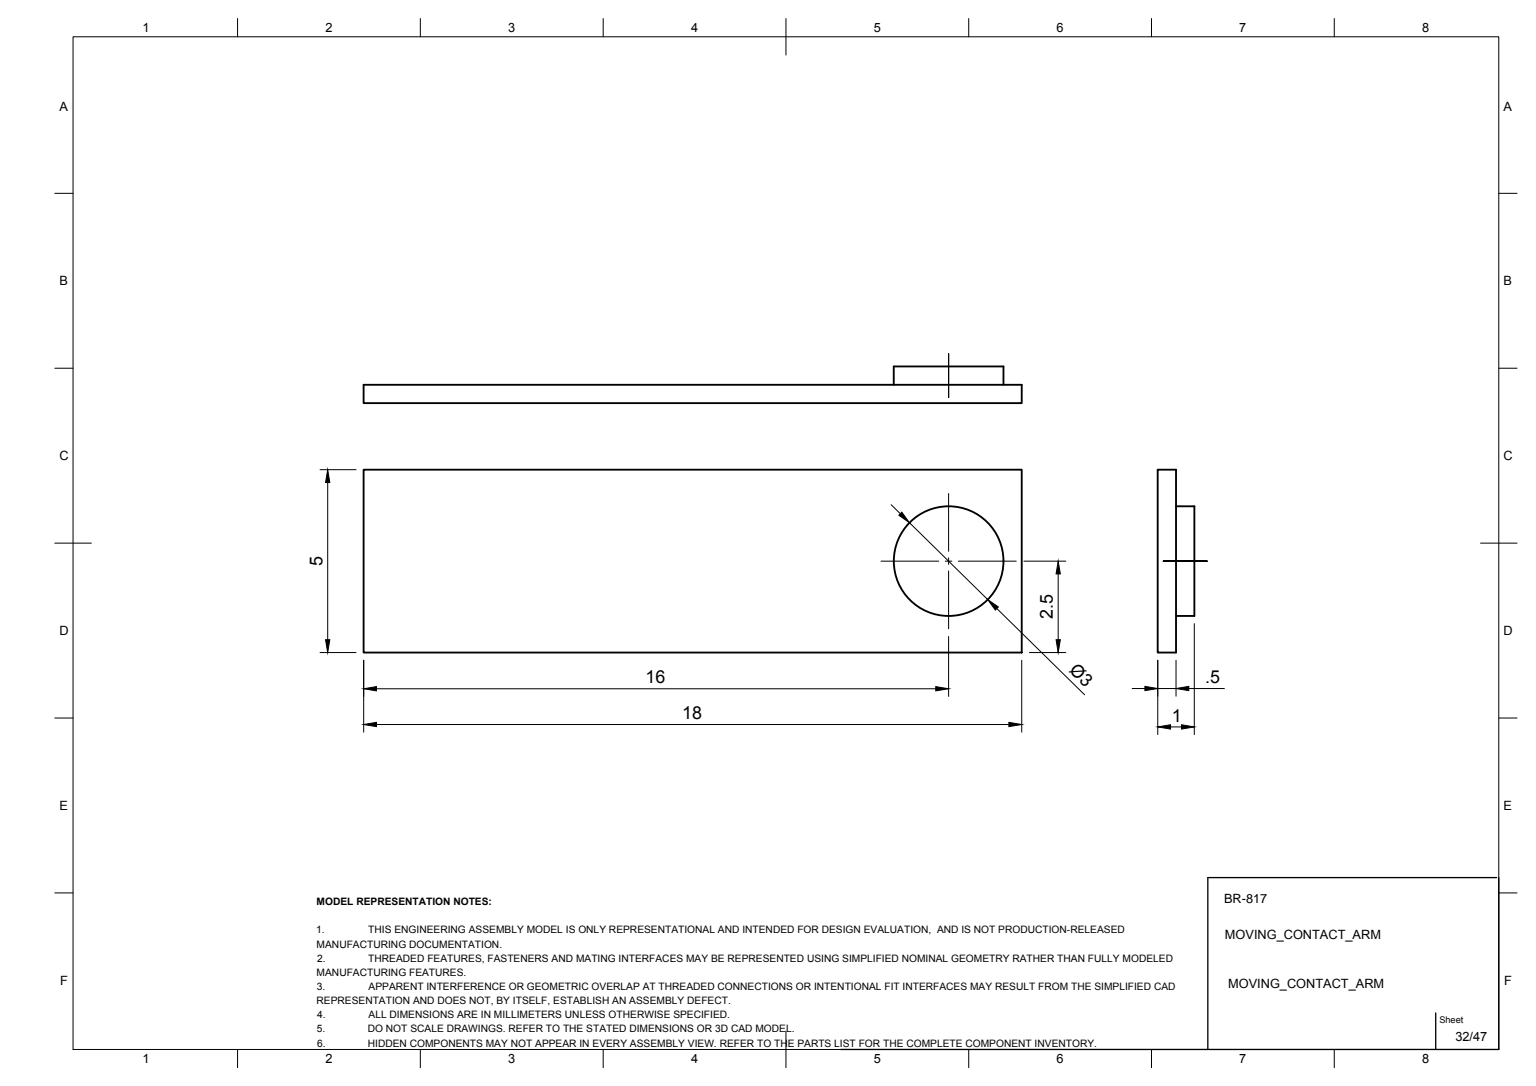
ISO-10303-21;
HEADER;
FILE_DESCRIPTION((''),'2;1');
FILE_NAME('MOVING_CONTACT_ARM.step','2026-10-01T22:07:29-07:00',(''),(''),'','','');
FILE_SCHEMA (('AUTOMOTIVE_DESIGN { 1 0 10303 214 3 1 1 }'));
ENDSEC;
DATA;
#10=MECHANICAL_DESIGN_GEOMETRIC_PRESENTATION_REPRESENTATION('',(#564),#15484);
#494=SHAPE_REPRESENTATION_RELATIONSHIP('SRR','None',#15644,#529) ;
#529=ADVANCED_BREP_SHAPE_REPRESENTATION('',(#605),#15468) ;
#564=STYLED_ITEM('',(#15834),#605) ;
#605=MANIFOLD_SOLID_BREP('MOVING_CONTACT_ARM',#8275) ;
#756=CYLINDRICAL_SURFACE('',#9515,0.15) ;
#875=FACE_BOUND('',#2272,.T.) ;
#1219=CIRCLE('',#9516,0.15) ;
#1220=CIRCLE('',#9517,0.15) ;
#1704=FACE_OUTER_BOUND('',#2269,.T.) ;
#1705=FACE_OUTER_BOUND('',#2270,.T.) ;
#1706=FACE_OUTER_BOUND('',#2271,.T.) ;
#1707=FACE_OUTER_BOUND('',#2273,.T.) ;
#1708=FACE_OUTER_BOUND('',#2274,.T.) ;
#1709=FACE_OUTER_BOUND('',#2275,.T.) ;
#1710=FACE_OUTER_BOUND('',#2276,.T.) ;
#1711=FACE_OUTER_BOUND('',#2277,.T.) ;
#2269=EDGE_LOOP('',(#6843,#6844,#6845,#6846)) ;
#2270=EDGE_LOOP('',(#6847)) ;
#2271=EDGE_LOOP('',(#6848,#6849,#6850,#6851)) ;
#2272=EDGE_LOOP('',(#6852)) ;
#2273=EDGE_LOOP('',(#6853,#6854,#6855,#6856)) ;
#2274=EDGE_LOOP('',(#6857,#6858,#6859,#6860)) ;
#2275=EDGE_LOOP('',(#6861,#6862,#6863,#6864)) ;
#2276=EDGE_LOOP('',(#6865,#6866,#6867,#6868)) ;
#2277=EDGE_LOOP('',(#6869,#6870,#6871,#6872)) ;
#2771=LINE('',#14620,#3245) ;
#2772=LINE('',#14626,#3246) ;
#2773=LINE('',#14628,#3247) ;
#2774=LINE('',#14630,#3248) ;
#2775=LINE('',#14631,#3249) ;
#2776=LINE('',#14635,#3250) ;
#2777=LINE('',#14637,#3251) ;
#2778=LINE('',#14639,#3252) ;
#2779=LINE('',#14640,#3253) ;
#2780=LINE('',#14642,#3254) ;
#2781=LINE('',#14643,#3255) ;
#2782=LINE('',#14645,#3256) ;
#2783=LINE('',#14647,#3257) ;
#3245=VECTOR('',#11926,0.15) ;
#3246=VECTOR('',#11933,1.) ;
#3247=VECTOR('',#11934,1.) ;
#3248=VECTOR('',#11935,1.) ;
#3249=VECTOR('',#11936,1.) ;
#3250=VECTOR('',#11939,1.) ;
#3251=VECTOR('',#11940,1.) ;
#3252=VECTOR('',#11941,1.) ;
#3253=VECTOR('',#11942,1.) ;
#3254=VECTOR('',#11945,1.) ;
#3255=VECTOR('',#11946,1.) ;
#3256=VECTOR('',#11949,1.) ;
#3257=VECTOR('',#11952,1.) ;
#3911=VERTEX_POINT('',#14617) ;
#3912=VERTEX_POINT('',#14619) ;
#3913=VERTEX_POINT('',#14624) ;
#3914=VERTEX_POINT('',#14625) ;
#3915=VERTEX_POINT('',#14627) ;
#3916=VERTEX_POINT('',#14629) ;
#3917=VERTEX_POINT('',#14633) ;
#3918=VERTEX_POINT('',#14634) ;
#3919=VERTEX_POINT('',#14636) ;
#3920=VERTEX_POINT('',#14638) ;
#4926=EDGE_CURVE('',#3911,#3911,#1219,.T.) ;
#4927=EDGE_CURVE('',#3911,#3912,#2771,.T.) ;
#4928=EDGE_CURVE('',#3912,#3912,#1220,.T.) ;
#4929=EDGE_CURVE('',#3913,#3914,#2772,.T.) ;
#4930=EDGE_CURVE('',#3914,#3915,#2773,.T.) ;
#4931=EDGE_CURVE('',#3915,#3916,#2774,.T.) ;
#4932=EDGE_CURVE('',#3916,#3913,#2775,.T.) ;
#4933=EDGE_CURVE('',#3917,#3918,#2776,.T.) ;
#4934=EDGE_CURVE('',#3918,#3919,#2777,.T.) ;
#4935=EDGE_CURVE('',#3919,#3920,#2778,.T.) ;
#4936=EDGE_CURVE('',#3920,#3917,#2779,.T.) ;
#4937=EDGE_CURVE('',#3916,#3919,#2780,.T.) ;
#4938=EDGE_CURVE('',#3913,#3918,#2781,.T.) ;
#4939=EDGE_CURVE('',#3915,#3920,#2782,.T.) ;
#4940=EDGE_CURVE('',#3914,#3917,#2783,.T.) ;
#6843=ORIENTED_EDGE('',*,*,#4926,.F.) ;
#6844=ORIENTED_EDGE('',*,*,#4927,.T.) ;
#6845=ORIENTED_EDGE('',*,*,#4928,.F.) ;
#6846=ORIENTED_EDGE('',*,*,#4927,.F.) ;
#6847=ORIENTED_EDGE('',*,*,#4926,.T.) ;
#6848=ORIENTED_EDGE('',*,*,#4929,.T.) ;
#6849=ORIENTED_EDGE('',*,*,#4930,.T.) ;
#6850=ORIENTED_EDGE('',*,*,#4931,.T.) ;
#6851=ORIENTED_EDGE('',*,*,#4932,.T.) ;
#6852=ORIENTED_EDGE('',*,*,#4928,.T.) ;
#6853=ORIENTED_EDGE('',*,*,#4933,.T.) ;
#6854=ORIENTED_EDGE('',*,*,#4934,.T.) ;
#6855=ORIENTED_EDGE('',*,*,#4935,.T.) ;
#6856=ORIENTED_EDGE('',*,*,#4936,.T.) ;
#6857=ORIENTED_EDGE('',*,*,#4937,.T.) ;
#6858=ORIENTED_EDGE('',*,*,#4934,.F.) ;
#6859=ORIENTED_EDGE('',*,*,#4938,.F.) ;
#6860=ORIENTED_EDGE('',*,*,#4932,.F.) ;
#6861=ORIENTED_EDGE('',*,*,#4939,.T.) ;
#6862=ORIENTED_EDGE('',*,*,#4935,.F.) ;
#6863=ORIENTED_EDGE('',*,*,#4937,.F.) ;
#6864=ORIENTED_EDGE('',*,*,#4931,.F.) ;
#6865=ORIENTED_EDGE('',*,*,#4940,.T.) ;
#6866=ORIENTED_EDGE('',*,*,#4936,.F.) ;
#6867=ORIENTED_EDGE('',*,*,#4939,.F.) ;
#6868=ORIENTED_EDGE('',*,*,#4930,.F.) ;
#6869=ORIENTED_EDGE('',*,*,#4938,.T.) ;
#6870=ORIENTED_EDGE('',*,*,#4933,.F.) ;
#6871=ORIENTED_EDGE('',*,*,#4940,.F.) ;
#6872=ORIENTED_EDGE('',*,*,#4929,.F.) ;
#7678=PLANE('',#9518) ;
#7679=PLANE('',#9519) ;
#7680=PLANE('',#9520) ;
#7681=PLANE('',#9521) ;
#7682=PLANE('',#9522) ;
#7683=PLANE('',#9523) ;
#7684=PLANE('',#9524) ;
#8091=ADVANCED_FACE('',(#1704),#756,.T.) ;
#8092=ADVANCED_FACE('',(#1705),#7678,.T.) ;
#8093=ADVANCED_FACE('',(#1706,#875),#7679,.T.) ;
#8094=ADVANCED_FACE('',(#1707),#7680,.F.) ;
#8095=ADVANCED_FACE('',(#1708),#7681,.F.) ;
#8096=ADVANCED_FACE('',(#1709),#7682,.F.) ;
#8097=ADVANCED_FACE('',(#1710),#7683,.F.) ;
#8098=ADVANCED_FACE('',(#1711),#7684,.F.) ;
#8275=CLOSED_SHELL('',(#8091,#8092,#8093,#8094,#8095,#8096,#8097,#8098)) ;
#9514=AXIS2_PLACEMENT_3D('',#14615,#11920,#11921) ;
#9515=AXIS2_PLACEMENT_3D('',#14616,#11922,#11923) ;
#9516=AXIS2_PLACEMENT_3D('',#14618,#11924,#11925) ;
#9517=AXIS2_PLACEMENT_3D('',#14621,#11927,#11928) ;
#9518=AXIS2_PLACEMENT_3D('',#14622,#11929,#11930) ;
#9519=AXIS2_PLACEMENT_3D('',#14623,#11931,#11932) ;
#9520=AXIS2_PLACEMENT_3D('',#14632,#11937,#11938) ;
#9521=AXIS2_PLACEMENT_3D('',#14641,#11943,#11944) ;
#9522=AXIS2_PLACEMENT_3D('',#14644,#11947,#11948) ;
#9523=AXIS2_PLACEMENT_3D('',#14646,#11950,#11951) ;
#9524=AXIS2_PLACEMENT_3D('',#14648,#11953,#11954) ;
#11920=DIRECTION('axis',(0.,0.,1.)) ;
#11921=DIRECTION('refdir',(1.,0.,0.)) ;
#11922=DIRECTION('center_axis',(0.,0.,1.)) ;
#11923=DIRECTION('ref_axis',(1.,0.,0.)) ;
#11924=DIRECTION('center_axis',(0.,0.,1.)) ;
#11925=DIRECTION('ref_axis',(1.,0.,0.)) ;
#11926=DIRECTION('',(0.,0.,-1.)) ;
#11927=DIRECTION('center_axis',(0.,0.,-1.)) ;
#11928=DIRECTION('ref_axis',(1.,0.,0.)) ;
#11929=DIRECTION('center_axis',(0.,0.,1.)) ;
#11930=DIRECTION('ref_axis',(1.,0.,0.)) ;
#11931=DIRECTION('center_axis',(0.,0.,1.)) ;
#11932=DIRECTION('ref_axis',(1.,0.,0.)) ;
#11933=DIRECTION('',(0.,1.,0.)) ;
#11934=DIRECTION('',(-1.,0.,0.)) ;
#11935=DIRECTION('',(0.,-1.,0.)) ;
#11936=DIRECTION('',(1.,0.,0.)) ;
#11937=DIRECTION('center_axis',(0.,0.,1.)) ;
#11938=DIRECTION('ref_axis',(1.,0.,0.)) ;
#11939=DIRECTION('',(0.,-1.,0.)) ;
#11940=DIRECTION('',(-1.,0.,0.)) ;
#11941=DIRECTION('',(0.,1.,0.)) ;
#11942=DIRECTION('',(1.,0.,0.)) ;
#11943=DIRECTION('center_axis',(0.,1.,0.)) ;
#11944=DIRECTION('ref_axis',(0.,0.,1.)) ;
#11945=DIRECTION('',(0.,0.,-1.)) ;
#11946=DIRECTION('',(0.,0.,-1.)) ;
#11947=DIRECTION('center_axis',(1.,0.,0.)) ;
#11948=DIRECTION('ref_axis',(0.,0.,-1.)) ;
#11949=DIRECTION('',(0.,0.,-1.)) ;
#11950=DIRECTION('center_axis',(0.,-1.,0.)) ;
#11951=DIRECTION('ref_axis',(0.,0.,-1.)) ;
#11952=DIRECTION('',(0.,0.,-1.)) ;
#11953=DIRECTION('center_axis',(-1.,0.,0.)) ;
#11954=DIRECTION('ref_axis',(0.,0.,1.)) ;
#14615=CARTESIAN_POINT('',(0.,0.,0.)) ;
#14616=CARTESIAN_POINT('Origin',(-1.1,-1.75,0.875)) ;
#14617=CARTESIAN_POINT('',(-1.25,-1.75,0.9)) ;
#14618=CARTESIAN_POINT('Origin',(-1.1,-1.75,0.9)) ;
#14619=CARTESIAN_POINT('',(-1.25,-1.75,0.85)) ;
#14620=CARTESIAN_POINT('',(-1.25,-1.75,0.875)) ;
#14621=CARTESIAN_POINT('Origin',(-1.1,-1.75,0.85)) ;
#14622=CARTESIAN_POINT('Origin',(-1.1,-1.75,0.9)) ;
#14623=CARTESIAN_POINT('Origin',(-1.8,-1.75,0.85)) ;
#14624=CARTESIAN_POINT('',(-0.9,-2.,0.85)) ;
#14625=CARTESIAN_POINT('',(-0.9,-1.5,0.85)) ;
#14626=CARTESIAN_POINT('',(-0.9,-1.75,0.85)) ;
#14627=CARTESIAN_POINT('',(-2.7,-1.5,0.85)) ;
#14628=CARTESIAN_POINT('',(-1.8,-1.5,0.85)) ;
#14629=CARTESIAN_POINT('',(-2.7,-2.,0.85)) ;
#14630=CARTESIAN_POINT('',(-2.7,-1.75,0.85)) ;
#14631=CARTESIAN_POINT('',(-1.8,-2.,0.85)) ;
#14632=CARTESIAN_POINT('Origin',(-1.8,-1.75,0.8)) ;
#14633=CARTESIAN_POINT('',(-0.9,-1.5,0.8)) ;
#14634=CARTESIAN_POINT('',(-0.9,-2.,0.8)) ;
#14635=CARTESIAN_POINT('',(-0.9,-1.75,0.8)) ;
#14636=CARTESIAN_POINT('',(-2.7,-2.,0.8)) ;
#14637=CARTESIAN_POINT('',(-1.8,-2.,0.8)) ;
#14638=CARTESIAN_POINT('',(-2.7,-1.5,0.8)) ;
#14639=CARTESIAN_POINT('',(-2.7,-1.75,0.8)) ;
#14640=CARTESIAN_POINT('',(-1.8,-1.5,0.8)) ;
#14641=CARTESIAN_POINT('Origin',(-1.8,-2.,0.825)) ;
#14642=CARTESIAN_POINT('',(-2.7,-2.,0.825)) ;
#14643=CARTESIAN_POINT('',(-0.9,-2.,0.825)) ;
#14644=CARTESIAN_POINT('Origin',(-2.7,-1.75,0.825)) ;
#14645=CARTESIAN_POINT('',(-2.7,-1.5,0.825)) ;
#14646=CARTESIAN_POINT('Origin',(-1.8,-1.5,0.825)) ;
#14647=CARTESIAN_POINT('',(-0.9,-1.5,0.825)) ;
#14648=CARTESIAN_POINT('Origin',(-0.9,-1.75,0.825)) ;
#15425=UNCERTAINTY_MEASURE_WITH_UNIT(LENGTH_MEASURE(0.001),#15485,
'DISTANCE_ACCURACY_VALUE',
'Maximum model space distance between geometric entities at asserted c
onnectivities') ;
#15441=UNCERTAINTY_MEASURE_WITH_UNIT(LENGTH_MEASURE(0.001),#15485,
'DISTANCE_ACCURACY_VALUE',
'Maximum model space distance between geometric entities at asserted c
onnectivities') ;
#15468=(
GEOMETRIC_REPRESENTATION_CONTEXT(3)
GLOBAL_UNCERTAINTY_ASSIGNED_CONTEXT((#15425))
GLOBAL_UNIT_ASSIGNED_CONTEXT((#15485,#15487,#15488))
REPRESENTATION_CONTEXT('','3D')
) ;
#15484=(
GEOMETRIC_REPRESENTATION_CONTEXT(3)
GLOBAL_UNCERTAINTY_ASSIGNED_CONTEXT((#15441))
GLOBAL_UNIT_ASSIGNED_CONTEXT((#15485,#15487,#15488))
REPRESENTATION_CONTEXT('','3D')
) ;
#15485=(
LENGTH_UNIT()
NAMED_UNIT(*)
SI_UNIT(.CENTI.,.METRE.)
) ;
#15487=(
NAMED_UNIT(*)
PLANE_ANGLE_UNIT()
SI_UNIT($,.RADIAN.)
) ;
#15488=(
NAMED_UNIT(*)
SI_UNIT($,.STERADIAN.)
SOLID_ANGLE_UNIT()
) ;
#15515=SHAPE_DEFINITION_REPRESENTATION(#15572,#15644) ;
#15572=PRODUCT_DEFINITION_SHAPE('',$,#15687) ;
#15644=SHAPE_REPRESENTATION('',(#9514),#15468) ;
#15660=PRODUCT_DEFINITION_CONTEXT('part definition',#15788,'design') ;
#15687=PRODUCT_DEFINITION('MOVING_CONTACT_ARM',
'MOVING_CONTACT_ARM',#15729,#15660) ;
#15729=PRODUCT_DEFINITION_FORMATION('',$,#15816) ;
#15788=APPLICATION_CONTEXT(
'Core Data for Automotive Mechanical Design Process') ;
#15789=PRODUCT_CONTEXT('part definition',#15788,'mechanical') ;
#15816=PRODUCT('MOVING_CONTACT_ARM','MOVING_CONTACT_ARM',$,(#15789)) ;
#15834=PRESENTATION_STYLE_ASSIGNMENT((#15846)) ;
#15846=SURFACE_STYLE_USAGE(.BOTH.,#15858) ;
#15858=SURFACE_SIDE_STYLE('',(#15870)) ;
#15870=SURFACE_STYLE_FILL_AREA(#15882) ;
#15882=FILL_AREA_STYLE('Brass - Polished',(#15894)) ;
#15894=FILL_AREA_STYLE_COLOUR('Brass - Polished',#15906) ;
#15906=COLOUR_RGB('Brass - Polished', 0.08235294, 0.09019608, 0.10196078) ;
ENDSEC;
END-ISO-10303-21;
